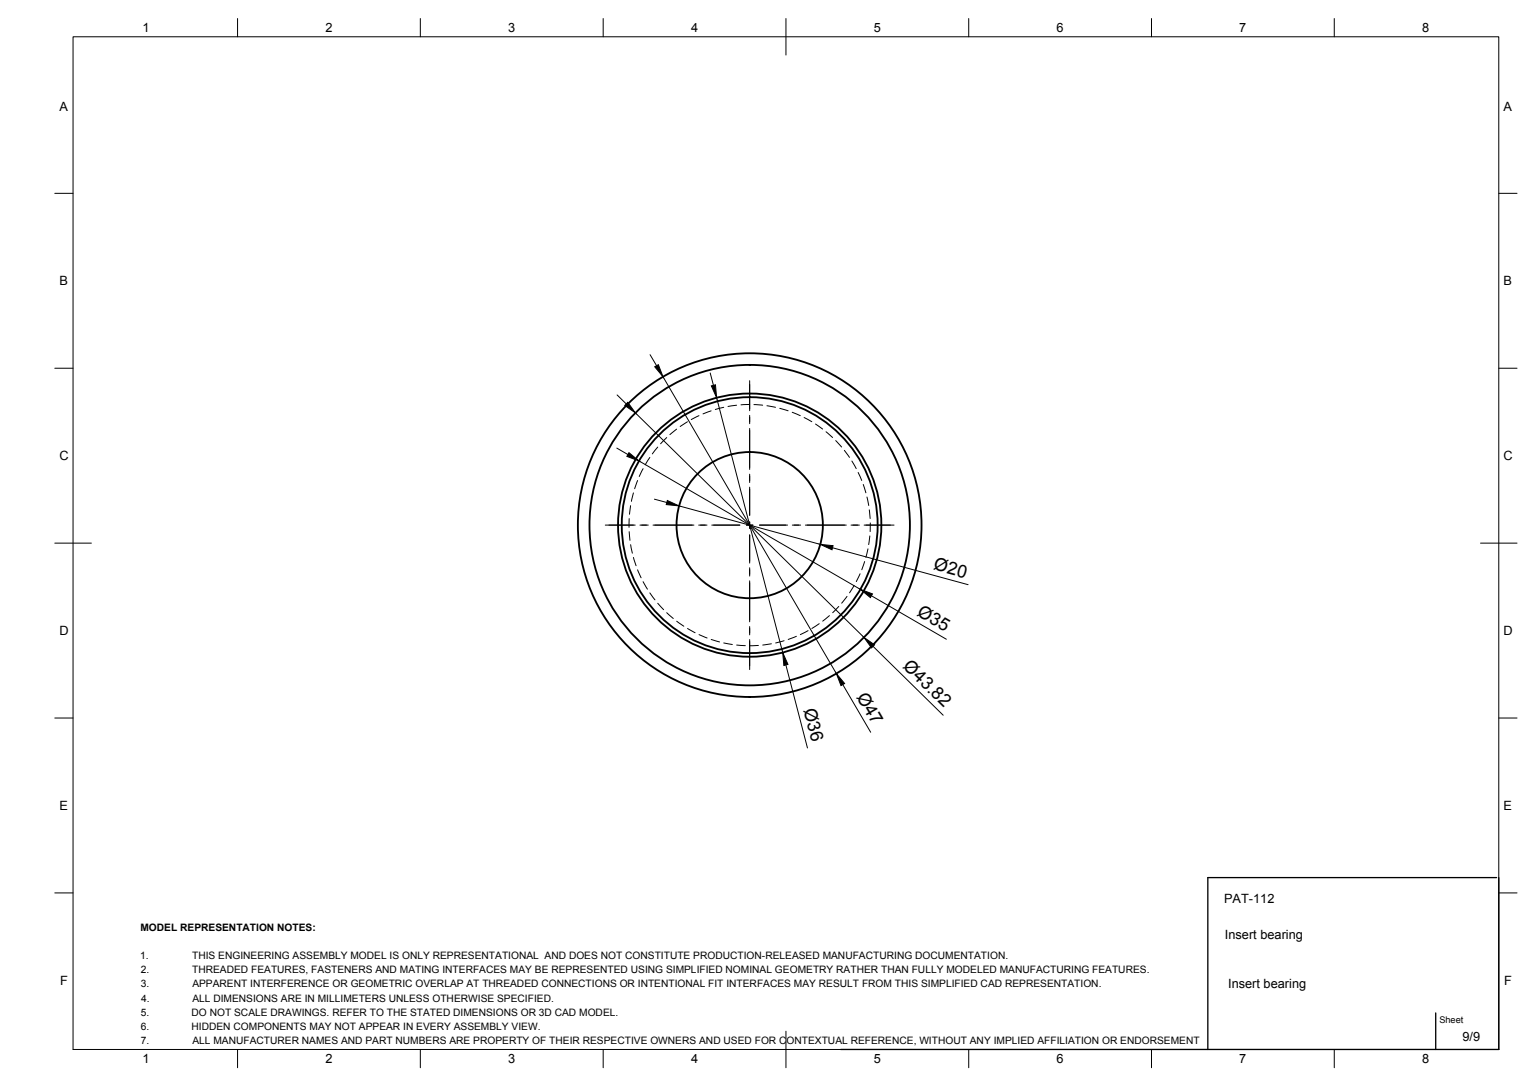
ISO-10303-21;
HEADER;
/* Generated by software containing ST-Developer
 * from STEP Tools, Inc. (www.steptools.com) 
 */

FILE_DESCRIPTION(
/* description */ ('PAT-112'),
/* implementation_level */ '2;1');

FILE_NAME(
/* name */ 'Insert bearing.step',
/* time_stamp */ '2026-11-15T15:25:42-08:00',
/* author */ (''),
/* organization */ (''),
/* preprocessor_version */ 'ST-DEVELOPER v20.2',
/* originating_system */ 'Autodesk Translation Framework v15.17.0.0',
/* authorisation */ '');

FILE_SCHEMA (('AUTOMOTIVE_DESIGN { 1 0 10303 214 3 1 1 }'));
ENDSEC;

DATA;
#10=MECHANICAL_DESIGN_GEOMETRIC_PRESENTATION_REPRESENTATION('',(#107,#108),#2277);
#90=SPHERICAL_SURFACE('',#1416,2.35);
#93=SHAPE_REPRESENTATION_RELATIONSHIP('SRR','None',#2322,#100);
#100=ADVANCED_BREP_SHAPE_REPRESENTATION('',(#115,#116),#2272);
#107=STYLED_ITEM('',(#2369),#115);
#108=STYLED_ITEM('',(#2369),#116);
#115=MANIFOLD_SOLID_BREP('Body1',#1259);
#116=MANIFOLD_SOLID_BREP('Body2',#1260);
#134=FACE_BOUND('',#329,.T.);
#135=FACE_BOUND('',#331,.T.);
#136=FACE_BOUND('',#332,.T.);
#137=FACE_BOUND('',#334,.T.);
#138=FACE_BOUND('',#337,.T.);
#139=FACE_BOUND('',#339,.T.);
#140=FACE_BOUND('',#342,.T.);
#175=PLANE('',#1414);
#176=PLANE('',#1419);
#177=PLANE('',#1423);
#178=PLANE('',#1425);
#179=PLANE('',#1429);
#236=FACE_OUTER_BOUND('',#327,.T.);
#237=FACE_OUTER_BOUND('',#328,.T.);
#238=FACE_OUTER_BOUND('',#330,.T.);
#239=FACE_OUTER_BOUND('',#333,.T.);
#240=FACE_OUTER_BOUND('',#335,.T.);
#241=FACE_OUTER_BOUND('',#336,.T.);
#242=FACE_OUTER_BOUND('',#338,.T.);
#243=FACE_OUTER_BOUND('',#340,.T.);
#244=FACE_OUTER_BOUND('',#341,.T.);
#245=FACE_OUTER_BOUND('',#343,.T.);
#327=EDGE_LOOP('',(#1036,#1037,#1038,#1039));
#328=EDGE_LOOP('',(#1040));
#329=EDGE_LOOP('',(#1041));
#330=EDGE_LOOP('',(#1042,#1043));
#331=EDGE_LOOP('',(#1044));
#332=EDGE_LOOP('',(#1045));
#333=EDGE_LOOP('',(#1046));
#334=EDGE_LOOP('',(#1047));
#335=EDGE_LOOP('',(#1048,#1049,#1050,#1051));
#336=EDGE_LOOP('',(#1052));
#337=EDGE_LOOP('',(#1053));
#338=EDGE_LOOP('',(#1054));
#339=EDGE_LOOP('',(#1055));
#340=EDGE_LOOP('',(#1056,#1057,#1058,#1059));
#341=EDGE_LOOP('',(#1060));
#342=EDGE_LOOP('',(#1061));
#343=EDGE_LOOP('',(#1062,#1063,#1064,#1065));
#439=LINE('',#2098,#534);
#440=LINE('',#2114,#535);
#441=LINE('',#2125,#536);
#442=LINE('',#2130,#537);
#534=VECTOR('',#1700,1.8);
#535=VECTOR('',#1719,1.65);
#536=VECTOR('',#1734,1.75);
#537=VECTOR('',#1741,1.);
#590=CIRCLE('',#1412,1.8);
#591=CIRCLE('',#1413,1.8);
#592=CIRCLE('',#1415,2.19089023002066);
#593=CIRCLE('',#1417,2.35);
#594=CIRCLE('',#1418,2.19089023002066);
#595=CIRCLE('',#1421,1.65);
#596=CIRCLE('',#1422,1.65);
#597=CIRCLE('',#1424,1.);
#598=CIRCLE('',#1426,1.75);
#599=CIRCLE('',#1428,1.75);
#600=CIRCLE('',#1430,1.);
#677=VERTEX_POINT('',#2095);
#678=VERTEX_POINT('',#2097);
#679=VERTEX_POINT('',#2101);
#680=VERTEX_POINT('',#2104);
#681=VERTEX_POINT('',#2105);
#682=VERTEX_POINT('',#2107);
#683=VERTEX_POINT('',#2111);
#684=VERTEX_POINT('',#2113);
#685=VERTEX_POINT('',#2117);
#686=VERTEX_POINT('',#2120);
#687=VERTEX_POINT('',#2123);
#688=VERTEX_POINT('',#2127);
#804=EDGE_CURVE('',#677,#677,#590,.T.);
#805=EDGE_CURVE('',#677,#678,#439,.T.);
#806=EDGE_CURVE('',#678,#678,#591,.T.);
#807=EDGE_CURVE('',#679,#679,#592,.T.);
#808=EDGE_CURVE('',#680,#681,#593,.T.);
#809=EDGE_CURVE('',#682,#682,#594,.T.);
#810=EDGE_CURVE('',#683,#683,#595,.T.);
#811=EDGE_CURVE('',#683,#684,#440,.T.);
#812=EDGE_CURVE('',#684,#684,#596,.T.);
#813=EDGE_CURVE('',#685,#685,#597,.T.);
#814=EDGE_CURVE('',#686,#686,#598,.T.);
#815=EDGE_CURVE('',#687,#687,#599,.T.);
#816=EDGE_CURVE('',#687,#686,#441,.T.);
#817=EDGE_CURVE('',#688,#688,#600,.T.);
#818=EDGE_CURVE('',#685,#688,#442,.T.);
#1036=ORIENTED_EDGE('',*,*,#804,.F.);
#1037=ORIENTED_EDGE('',*,*,#805,.T.);
#1038=ORIENTED_EDGE('',*,*,#806,.T.);
#1039=ORIENTED_EDGE('',*,*,#805,.F.);
#1040=ORIENTED_EDGE('',*,*,#807,.F.);
#1041=ORIENTED_EDGE('',*,*,#804,.T.);
#1042=ORIENTED_EDGE('',*,*,#808,.T.);
#1043=ORIENTED_EDGE('',*,*,#808,.F.);
#1044=ORIENTED_EDGE('',*,*,#807,.T.);
#1045=ORIENTED_EDGE('',*,*,#809,.F.);
#1046=ORIENTED_EDGE('',*,*,#809,.T.);
#1047=ORIENTED_EDGE('',*,*,#806,.F.);
#1048=ORIENTED_EDGE('',*,*,#810,.F.);
#1049=ORIENTED_EDGE('',*,*,#811,.T.);
#1050=ORIENTED_EDGE('',*,*,#812,.T.);
#1051=ORIENTED_EDGE('',*,*,#811,.F.);
#1052=ORIENTED_EDGE('',*,*,#812,.F.);
#1053=ORIENTED_EDGE('',*,*,#813,.T.);
#1054=ORIENTED_EDGE('',*,*,#814,.F.);
#1055=ORIENTED_EDGE('',*,*,#810,.T.);
#1056=ORIENTED_EDGE('',*,*,#815,.F.);
#1057=ORIENTED_EDGE('',*,*,#816,.T.);
#1058=ORIENTED_EDGE('',*,*,#814,.T.);
#1059=ORIENTED_EDGE('',*,*,#816,.F.);
#1060=ORIENTED_EDGE('',*,*,#815,.T.);
#1061=ORIENTED_EDGE('',*,*,#817,.F.);
#1062=ORIENTED_EDGE('',*,*,#813,.F.);
#1063=ORIENTED_EDGE('',*,*,#818,.T.);
#1064=ORIENTED_EDGE('',*,*,#817,.T.);
#1065=ORIENTED_EDGE('',*,*,#818,.F.);
#1169=CYLINDRICAL_SURFACE('',#1411,1.8);
#1170=CYLINDRICAL_SURFACE('',#1420,1.65);
#1171=CYLINDRICAL_SURFACE('',#1427,1.75);
#1172=CYLINDRICAL_SURFACE('',#1431,1.);
#1219=ADVANCED_FACE('',(#236),#1169,.F.);
#1220=ADVANCED_FACE('',(#237,#134),#175,.T.);
#1221=ADVANCED_FACE('',(#238,#135,#136),#90,.T.);
#1222=ADVANCED_FACE('',(#239,#137),#176,.T.);
#1223=ADVANCED_FACE('',(#240),#1170,.T.);
#1224=ADVANCED_FACE('',(#241,#138),#177,.T.);
#1225=ADVANCED_FACE('',(#242,#139),#178,.T.);
#1226=ADVANCED_FACE('',(#243),#1171,.T.);
#1227=ADVANCED_FACE('',(#244,#140),#179,.T.);
#1228=ADVANCED_FACE('',(#245),#1172,.F.);
#1259=CLOSED_SHELL('',(#1219,#1220,#1221,#1222));
#1260=CLOSED_SHELL('',(#1223,#1224,#1225,#1226,#1227,#1228));
#1410=AXIS2_PLACEMENT_3D('',#2093,#1694,#1695);
#1411=AXIS2_PLACEMENT_3D('',#2094,#1696,#1697);
#1412=AXIS2_PLACEMENT_3D('',#2096,#1698,#1699);
#1413=AXIS2_PLACEMENT_3D('',#2099,#1701,#1702);
#1414=AXIS2_PLACEMENT_3D('',#2100,#1703,#1704);
#1415=AXIS2_PLACEMENT_3D('',#2102,#1705,#1706);
#1416=AXIS2_PLACEMENT_3D('',#2103,#1707,#1708);
#1417=AXIS2_PLACEMENT_3D('',#2106,#1709,#1710);
#1418=AXIS2_PLACEMENT_3D('',#2108,#1711,#1712);
#1419=AXIS2_PLACEMENT_3D('',#2109,#1713,#1714);
#1420=AXIS2_PLACEMENT_3D('',#2110,#1715,#1716);
#1421=AXIS2_PLACEMENT_3D('',#2112,#1717,#1718);
#1422=AXIS2_PLACEMENT_3D('',#2115,#1720,#1721);
#1423=AXIS2_PLACEMENT_3D('',#2116,#1722,#1723);
#1424=AXIS2_PLACEMENT_3D('',#2118,#1724,#1725);
#1425=AXIS2_PLACEMENT_3D('',#2119,#1726,#1727);
#1426=AXIS2_PLACEMENT_3D('',#2121,#1728,#1729);
#1427=AXIS2_PLACEMENT_3D('',#2122,#1730,#1731);
#1428=AXIS2_PLACEMENT_3D('',#2124,#1732,#1733);
#1429=AXIS2_PLACEMENT_3D('',#2126,#1735,#1736);
#1430=AXIS2_PLACEMENT_3D('',#2128,#1737,#1738);
#1431=AXIS2_PLACEMENT_3D('',#2129,#1739,#1740);
#1694=DIRECTION('axis',(0.,0.,1.));
#1695=DIRECTION('refdir',(1.,0.,0.));
#1696=DIRECTION('center_axis',(0.,-1.,0.));
#1697=DIRECTION('ref_axis',(1.,0.,0.));
#1698=DIRECTION('center_axis',(0.,-1.,0.));
#1699=DIRECTION('ref_axis',(1.,0.,0.));
#1700=DIRECTION('',(0.,-1.,0.));
#1701=DIRECTION('center_axis',(0.,-1.,0.));
#1702=DIRECTION('ref_axis',(1.,0.,0.));
#1703=DIRECTION('center_axis',(0.,1.,0.));
#1704=DIRECTION('ref_axis',(0.,0.,1.));
#1705=DIRECTION('center_axis',(0.,-1.,0.));
#1706=DIRECTION('ref_axis',(1.,0.,0.));
#1707=DIRECTION('center_axis',(1.22464679914735E-16,0.,1.));
#1708=DIRECTION('ref_axis',(1.,0.,-6.12323399573677E-17));
#1709=DIRECTION('center_axis',(1.22464679914735E-16,-1.,-7.49879891330929E-33));
#1710=DIRECTION('ref_axis',(-1.,-1.22464679914735E-16,6.12323399573677E-17));
#1711=DIRECTION('center_axis',(0.,-1.,0.));
#1712=DIRECTION('ref_axis',(1.,0.,0.));
#1713=DIRECTION('center_axis',(0.,-1.,0.));
#1714=DIRECTION('ref_axis',(0.,0.,-1.));
#1715=DIRECTION('center_axis',(0.,-1.,0.));
#1716=DIRECTION('ref_axis',(1.,0.,0.));
#1717=DIRECTION('center_axis',(0.,-1.,0.));
#1718=DIRECTION('ref_axis',(1.,0.,0.));
#1719=DIRECTION('',(0.,1.,0.));
#1720=DIRECTION('center_axis',(0.,-1.,0.));
#1721=DIRECTION('ref_axis',(1.,0.,0.));
#1722=DIRECTION('center_axis',(0.,1.,0.));
#1723=DIRECTION('ref_axis',(0.,0.,1.));
#1724=DIRECTION('center_axis',(0.,-1.,0.));
#1725=DIRECTION('ref_axis',(1.,0.,0.));
#1726=DIRECTION('center_axis',(0.,1.,0.));
#1727=DIRECTION('ref_axis',(0.,0.,1.));
#1728=DIRECTION('center_axis',(0.,-1.,0.));
#1729=DIRECTION('ref_axis',(1.,0.,0.));
#1730=DIRECTION('center_axis',(0.,-1.,0.));
#1731=DIRECTION('ref_axis',(1.,0.,0.));
#1732=DIRECTION('center_axis',(0.,-1.,0.));
#1733=DIRECTION('ref_axis',(1.,0.,0.));
#1734=DIRECTION('',(0.,1.,0.));
#1735=DIRECTION('center_axis',(0.,-1.,0.));
#1736=DIRECTION('ref_axis',(0.,0.,-1.));
#1737=DIRECTION('center_axis',(0.,-1.,0.));
#1738=DIRECTION('ref_axis',(1.,0.,0.));
#1739=DIRECTION('center_axis',(0.,-1.,0.));
#1740=DIRECTION('ref_axis',(1.,0.,0.));
#1741=DIRECTION('',(0.,-1.,0.));
#2093=CARTESIAN_POINT('',(0.,0.,0.));
#2094=CARTESIAN_POINT('Origin',(0.,0.,0.));
#2095=CARTESIAN_POINT('',(-1.8,0.85,-2.20436423846524E-16));
#2096=CARTESIAN_POINT('Origin',(0.,0.85,0.));
#2097=CARTESIAN_POINT('',(-1.8,-0.85,-2.20436423846524E-16));
#2098=CARTESIAN_POINT('',(-1.8,0.,-2.20436423846524E-16));
#2099=CARTESIAN_POINT('Origin',(0.,-0.85,0.));
#2100=CARTESIAN_POINT('Origin',(2.19089023002066,0.85,0.));
#2101=CARTESIAN_POINT('',(2.19089023002066,0.85,0.));
#2102=CARTESIAN_POINT('Origin',(0.,0.85,0.));
#2103=CARTESIAN_POINT('Origin',(3.99680288865056E-15,0.,0.));
#2104=CARTESIAN_POINT('',(3.99680288865056E-15,-1.76221774462768E-32,2.35));
#2105=CARTESIAN_POINT('',(3.70901089085093E-15,-1.76221774462768E-32,-2.35));
#2106=CARTESIAN_POINT('Origin',(3.99680288865056E-15,0.,0.));
#2107=CARTESIAN_POINT('',(2.19089023002066,-0.85,0.));
#2108=CARTESIAN_POINT('Origin',(0.,-0.85,0.));
#2109=CARTESIAN_POINT('Origin',(1.8,-0.85,0.));
#2110=CARTESIAN_POINT('Origin',(0.,1.55,0.));
#2111=CARTESIAN_POINT('',(-1.65,0.85,-2.02066721859313E-16));
#2112=CARTESIAN_POINT('Origin',(0.,0.85,0.));
#2113=CARTESIAN_POINT('',(-1.65,2.25,-2.02066721859313E-16));
#2114=CARTESIAN_POINT('',(-1.65,1.55,-2.02066721859313E-16));
#2115=CARTESIAN_POINT('Origin',(0.,2.25,0.));
#2116=CARTESIAN_POINT('Origin',(1.65,2.25,0.));
#2117=CARTESIAN_POINT('',(-1.,2.25,-1.22464679914735E-16));
#2118=CARTESIAN_POINT('Origin',(0.,2.25,0.));
#2119=CARTESIAN_POINT('Origin',(1.75,0.85,0.));
#2120=CARTESIAN_POINT('',(-1.75,0.85,-2.14313189850787E-16));
#2121=CARTESIAN_POINT('Origin',(0.,0.85,0.));
#2122=CARTESIAN_POINT('Origin',(0.,0.,0.));
#2123=CARTESIAN_POINT('',(-1.75,-0.85,-2.14313189850787E-16));
#2124=CARTESIAN_POINT('Origin',(0.,-0.85,0.));
#2125=CARTESIAN_POINT('',(-1.75,0.,-2.14313189850787E-16));
#2126=CARTESIAN_POINT('Origin',(1.,-0.85,0.));
#2127=CARTESIAN_POINT('',(-1.,-0.85,-1.22464679914735E-16));
#2128=CARTESIAN_POINT('Origin',(0.,-0.85,0.));
#2129=CARTESIAN_POINT('Origin',(0.,0.7,0.));
#2130=CARTESIAN_POINT('',(-1.,0.7,-1.22464679914735E-16));
#2262=UNCERTAINTY_MEASURE_WITH_UNIT(LENGTH_MEASURE(0.001),#2278,
'DISTANCE_ACCURACY_VALUE',
'Maximum model space distance between geometric entities at asserted c
onnectivities');
#2267=UNCERTAINTY_MEASURE_WITH_UNIT(LENGTH_MEASURE(0.001),#2278,
'DISTANCE_ACCURACY_VALUE',
'Maximum model space distance between geometric entities at asserted c
onnectivities');
#2272=(
GEOMETRIC_REPRESENTATION_CONTEXT(3)
GLOBAL_UNCERTAINTY_ASSIGNED_CONTEXT((#2262))
GLOBAL_UNIT_ASSIGNED_CONTEXT((#2278,#2280,#2281))
REPRESENTATION_CONTEXT('','3D')
);
#2277=(
GEOMETRIC_REPRESENTATION_CONTEXT(3)
GLOBAL_UNCERTAINTY_ASSIGNED_CONTEXT((#2267))
GLOBAL_UNIT_ASSIGNED_CONTEXT((#2278,#2280,#2281))
REPRESENTATION_CONTEXT('','3D')
);
#2278=(
LENGTH_UNIT()
NAMED_UNIT(*)
SI_UNIT(.CENTI.,.METRE.)
);
#2280=(
NAMED_UNIT(*)
PLANE_ANGLE_UNIT()
SI_UNIT($,.RADIAN.)
);
#2281=(
NAMED_UNIT(*)
SI_UNIT($,.STERADIAN.)
SOLID_ANGLE_UNIT()
);
#2286=SHAPE_DEFINITION_REPRESENTATION(#2295,#2322);
#2295=PRODUCT_DEFINITION_SHAPE('',$,#2332);
#2322=SHAPE_REPRESENTATION('',(#1410),#2272);
#2327=PRODUCT_DEFINITION_CONTEXT('part definition',#2356,'design');
#2332=PRODUCT_DEFINITION('Insert bearing','Insert bearing',#2341,#2327);
#2341=PRODUCT_DEFINITION_FORMATION('',$,#2362);
#2356=APPLICATION_CONTEXT(
'Core Data for Automotive Mechanical Design Process');
#2357=PRODUCT_CONTEXT('part definition',#2356,'mechanical');
#2362=PRODUCT('Insert bearing','Insert bearing','Insert bearing',(#2357));
#2369=PRESENTATION_STYLE_ASSIGNMENT((#2374));
#2374=SURFACE_STYLE_USAGE(.BOTH.,#2379);
#2379=SURFACE_SIDE_STYLE('',(#2384));
#2384=SURFACE_STYLE_FILL_AREA(#2389);
#2389=FILL_AREA_STYLE('Opaque(122,133,145)',(#2394));
#2394=FILL_AREA_STYLE_COLOUR('Opaque(122,133,145)',#2399);
#2399=COLOUR_RGB('Opaque(122,133,145)',0.47843137254902,0.52156862745098,
0.568627450980392);
ENDSEC;
END-ISO-10303-21;
